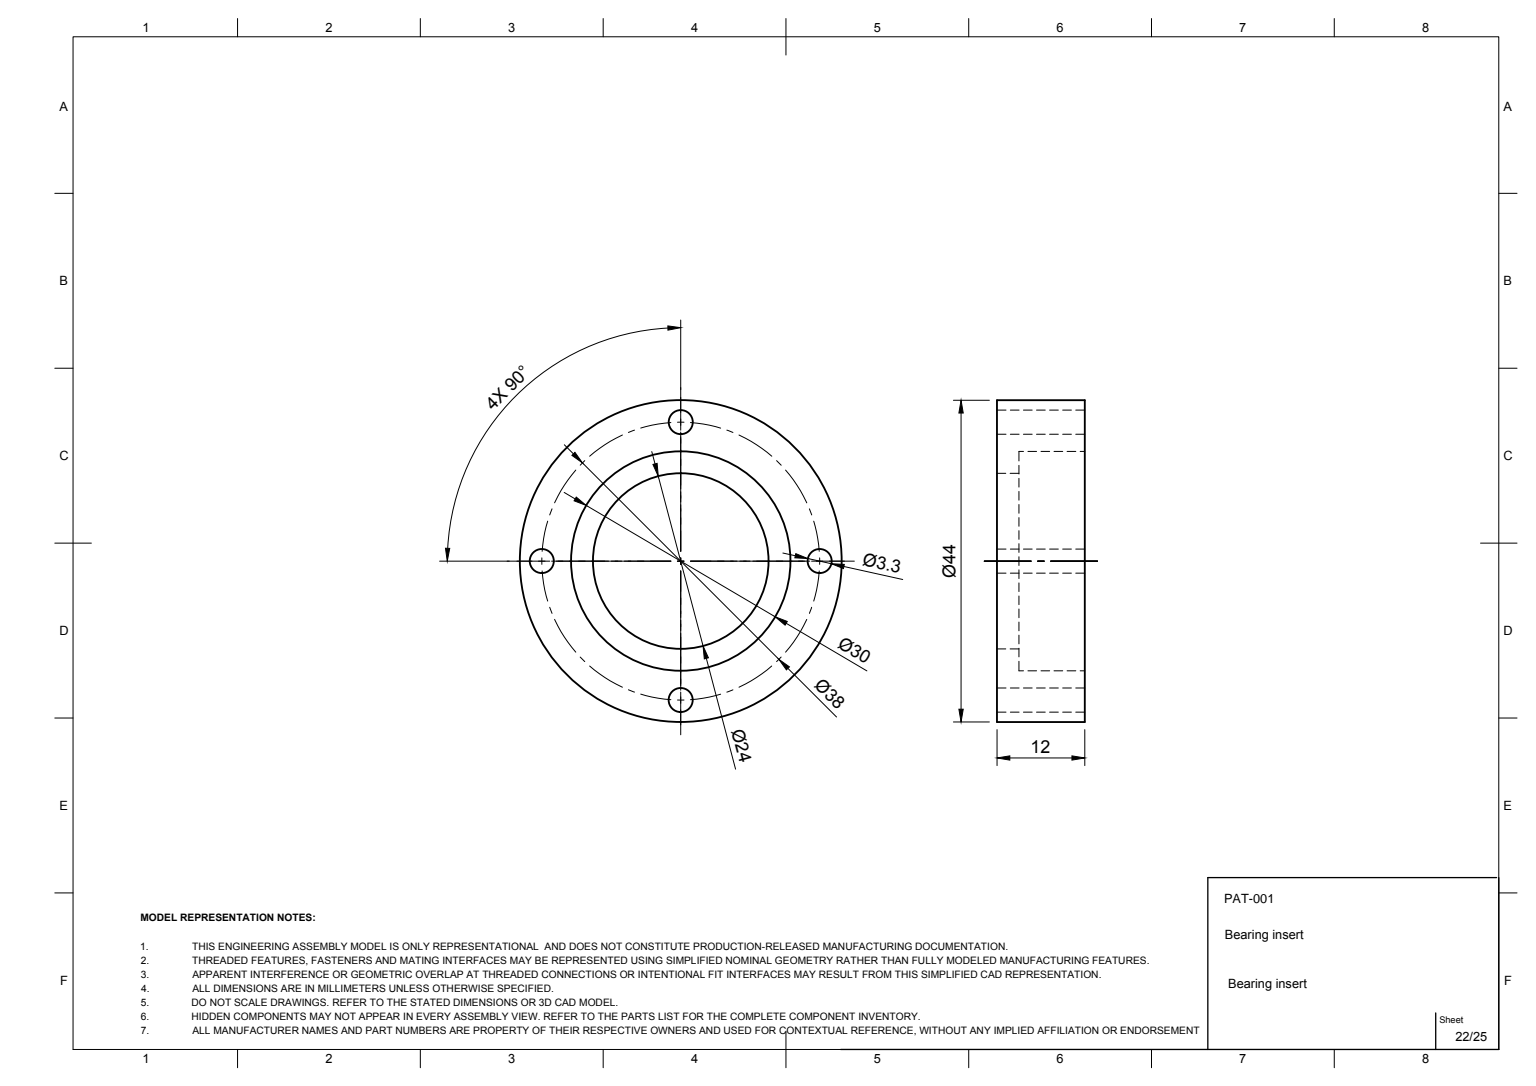
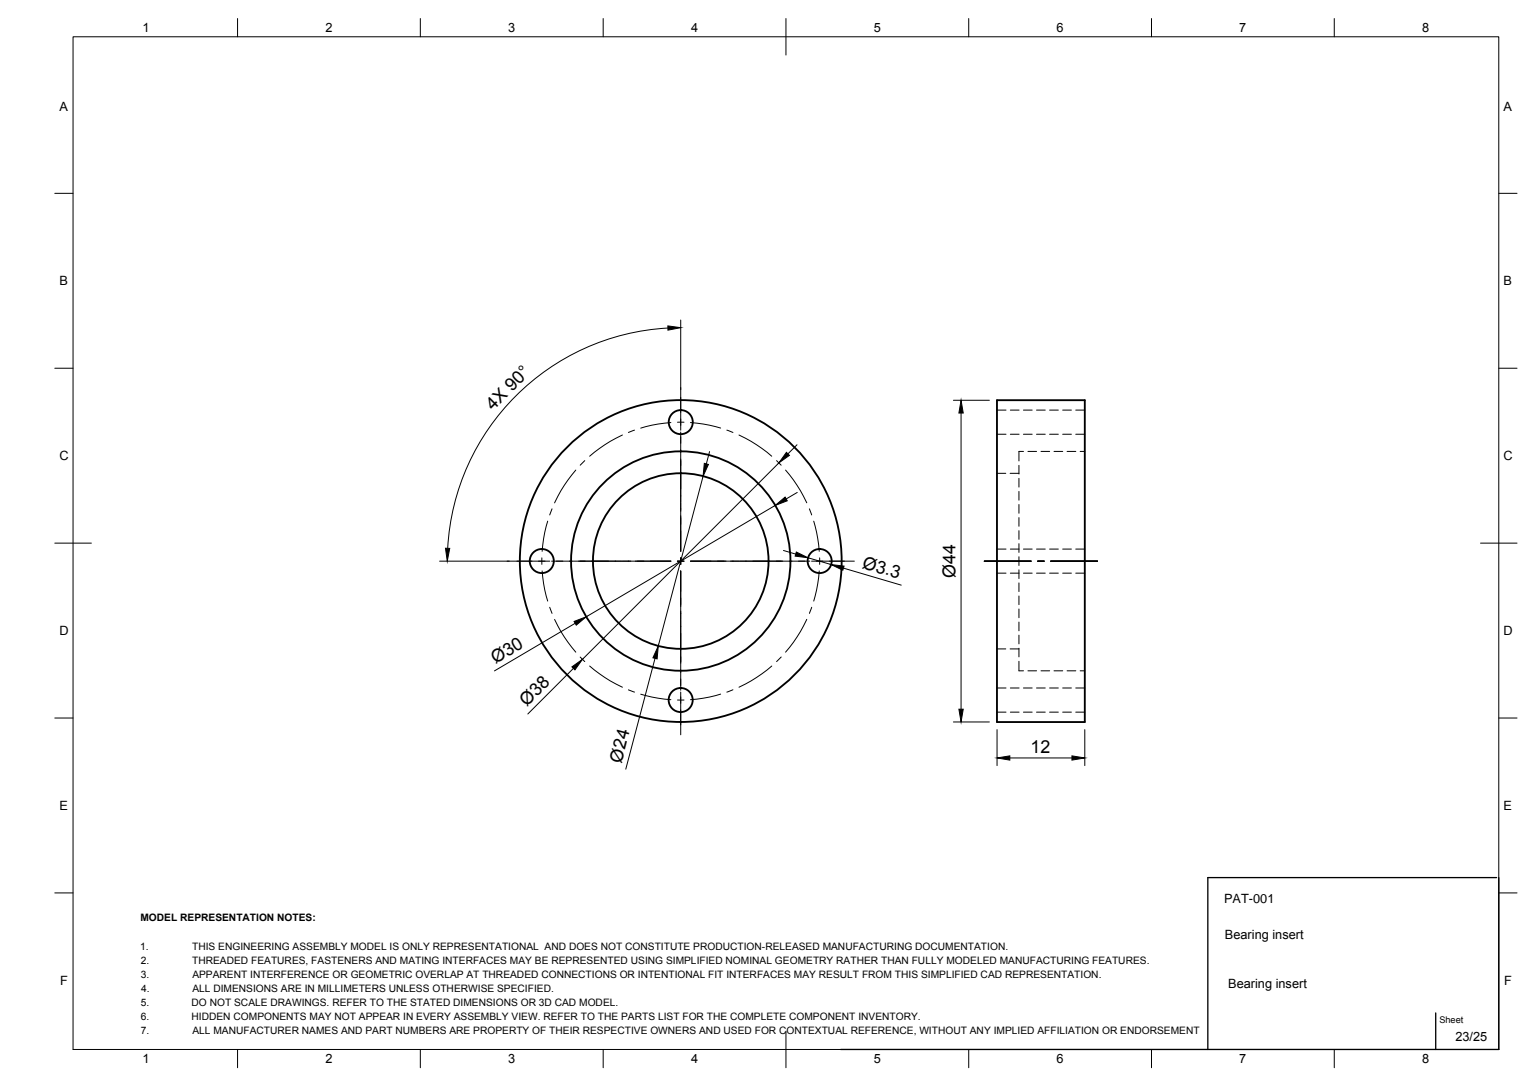
ISO-10303-21;
HEADER;
/* Generated by software containing ST-Developer
 * from STEP Tools, Inc. (www.steptools.com) 
 */

FILE_DESCRIPTION(
/* description */ ('PAT-001'),
/* implementation_level */ '2;1');

FILE_NAME(
/* name */ 'Bearing insert.step',
/* time_stamp */ '2026-10-29T17:07:15-07:00',
/* author */ (''),
/* organization */ (''),
/* preprocessor_version */ 'ST-DEVELOPER v20.2',
/* originating_system */ 'Autodesk Translation Framework v15.17.0.0',
/* authorisation */ '');

FILE_SCHEMA (('AUTOMOTIVE_DESIGN { 1 0 10303 214 3 1 1 }'));
ENDSEC;

DATA;
#10=MECHANICAL_DESIGN_GEOMETRIC_PRESENTATION_REPRESENTATION('',(#401),#9622);
#343=SHAPE_REPRESENTATION_RELATIONSHIP('SRR','None',#9768,#368);
#368=ADVANCED_BREP_SHAPE_REPRESENTATION('',(#433),#9617);
#401=STYLED_ITEM('',(#9962),#433);
#433=MANIFOLD_SOLID_BREP('Body1',#5227);
#493=FACE_BOUND('',#1320,.T.);
#494=FACE_BOUND('',#1324,.T.);
#495=FACE_BOUND('',#1325,.T.);
#496=FACE_BOUND('',#1326,.T.);
#497=FACE_BOUND('',#1327,.T.);
#498=FACE_BOUND('',#1328,.T.);
#499=FACE_BOUND('',#1330,.T.);
#500=FACE_BOUND('',#1331,.T.);
#501=FACE_BOUND('',#1332,.T.);
#502=FACE_BOUND('',#1333,.T.);
#503=FACE_BOUND('',#1334,.T.);
#694=PLANE('',#5963);
#695=PLANE('',#5970);
#696=PLANE('',#5971);
#962=FACE_OUTER_BOUND('',#1314,.T.);
#963=FACE_OUTER_BOUND('',#1315,.T.);
#964=FACE_OUTER_BOUND('',#1316,.T.);
#965=FACE_OUTER_BOUND('',#1317,.T.);
#966=FACE_OUTER_BOUND('',#1318,.T.);
#967=FACE_OUTER_BOUND('',#1319,.T.);
#968=FACE_OUTER_BOUND('',#1321,.T.);
#969=FACE_OUTER_BOUND('',#1322,.T.);
#970=FACE_OUTER_BOUND('',#1323,.T.);
#971=FACE_OUTER_BOUND('',#1329,.T.);
#1314=EDGE_LOOP('',(#4631,#4632,#4633,#4634));
#1315=EDGE_LOOP('',(#4635,#4636,#4637,#4638));
#1316=EDGE_LOOP('',(#4639,#4640,#4641,#4642));
#1317=EDGE_LOOP('',(#4643,#4644,#4645,#4646));
#1318=EDGE_LOOP('',(#4647,#4648,#4649,#4650));
#1319=EDGE_LOOP('',(#4651));
#1320=EDGE_LOOP('',(#4652));
#1321=EDGE_LOOP('',(#4653,#4654,#4655,#4656));
#1322=EDGE_LOOP('',(#4657,#4658,#4659,#4660));
#1323=EDGE_LOOP('',(#4661));
#1324=EDGE_LOOP('',(#4662));
#1325=EDGE_LOOP('',(#4663));
#1326=EDGE_LOOP('',(#4664));
#1327=EDGE_LOOP('',(#4665));
#1328=EDGE_LOOP('',(#4666));
#1329=EDGE_LOOP('',(#4667));
#1330=EDGE_LOOP('',(#4668));
#1331=EDGE_LOOP('',(#4669));
#1332=EDGE_LOOP('',(#4670));
#1333=EDGE_LOOP('',(#4671));
#1334=EDGE_LOOP('',(#4672));
#1757=LINE('',#9298,#2162);
#1758=LINE('',#9304,#2163);
#1759=LINE('',#9310,#2164);
#1760=LINE('',#9316,#2165);
#1761=LINE('',#9322,#2166);
#1762=LINE('',#9329,#2167);
#1763=LINE('',#9335,#2168);
#2162=VECTOR('',#7348,0.165);
#2163=VECTOR('',#7355,0.165);
#2164=VECTOR('',#7362,0.165);
#2165=VECTOR('',#7369,0.165);
#2166=VECTOR('',#7376,1.2);
#2167=VECTOR('',#7385,1.5);
#2168=VECTOR('',#7392,2.2);
#2368=CIRCLE('',#5949,0.165);
#2369=CIRCLE('',#5950,0.165);
#2370=CIRCLE('',#5952,0.165);
#2371=CIRCLE('',#5953,0.165);
#2372=CIRCLE('',#5955,0.165);
#2373=CIRCLE('',#5956,0.165);
#2374=CIRCLE('',#5958,0.165);
#2375=CIRCLE('',#5959,0.165);
#2376=CIRCLE('',#5961,1.2);
#2377=CIRCLE('',#5962,1.2);
#2378=CIRCLE('',#5964,1.5);
#2379=CIRCLE('',#5966,1.5);
#2380=CIRCLE('',#5968,2.2);
#2381=CIRCLE('',#5969,2.2);
#2798=VERTEX_POINT('',#9295);
#2799=VERTEX_POINT('',#9297);
#2800=VERTEX_POINT('',#9301);
#2801=VERTEX_POINT('',#9303);
#2802=VERTEX_POINT('',#9307);
#2803=VERTEX_POINT('',#9309);
#2804=VERTEX_POINT('',#9313);
#2805=VERTEX_POINT('',#9315);
#2806=VERTEX_POINT('',#9319);
#2807=VERTEX_POINT('',#9321);
#2808=VERTEX_POINT('',#9325);
#2809=VERTEX_POINT('',#9328);
#2810=VERTEX_POINT('',#9332);
#2811=VERTEX_POINT('',#9334);
#3419=EDGE_CURVE('',#2798,#2798,#2368,.T.);
#3420=EDGE_CURVE('',#2798,#2799,#1757,.T.);
#3421=EDGE_CURVE('',#2799,#2799,#2369,.T.);
#3422=EDGE_CURVE('',#2800,#2800,#2370,.T.);
#3423=EDGE_CURVE('',#2800,#2801,#1758,.T.);
#3424=EDGE_CURVE('',#2801,#2801,#2371,.T.);
#3425=EDGE_CURVE('',#2802,#2802,#2372,.T.);
#3426=EDGE_CURVE('',#2802,#2803,#1759,.T.);
#3427=EDGE_CURVE('',#2803,#2803,#2373,.T.);
#3428=EDGE_CURVE('',#2804,#2804,#2374,.T.);
#3429=EDGE_CURVE('',#2804,#2805,#1760,.T.);
#3430=EDGE_CURVE('',#2805,#2805,#2375,.T.);
#3431=EDGE_CURVE('',#2806,#2806,#2376,.T.);
#3432=EDGE_CURVE('',#2806,#2807,#1761,.T.);
#3433=EDGE_CURVE('',#2807,#2807,#2377,.T.);
#3434=EDGE_CURVE('',#2808,#2808,#2378,.T.);
#3435=EDGE_CURVE('',#2808,#2809,#1762,.T.);
#3436=EDGE_CURVE('',#2809,#2809,#2379,.T.);
#3437=EDGE_CURVE('',#2810,#2810,#2380,.T.);
#3438=EDGE_CURVE('',#2810,#2811,#1763,.T.);
#3439=EDGE_CURVE('',#2811,#2811,#2381,.T.);
#4631=ORIENTED_EDGE('',*,*,#3419,.F.);
#4632=ORIENTED_EDGE('',*,*,#3420,.T.);
#4633=ORIENTED_EDGE('',*,*,#3421,.F.);
#4634=ORIENTED_EDGE('',*,*,#3420,.F.);
#4635=ORIENTED_EDGE('',*,*,#3422,.F.);
#4636=ORIENTED_EDGE('',*,*,#3423,.T.);
#4637=ORIENTED_EDGE('',*,*,#3424,.F.);
#4638=ORIENTED_EDGE('',*,*,#3423,.F.);
#4639=ORIENTED_EDGE('',*,*,#3425,.F.);
#4640=ORIENTED_EDGE('',*,*,#3426,.T.);
#4641=ORIENTED_EDGE('',*,*,#3427,.F.);
#4642=ORIENTED_EDGE('',*,*,#3426,.F.);
#4643=ORIENTED_EDGE('',*,*,#3428,.F.);
#4644=ORIENTED_EDGE('',*,*,#3429,.T.);
#4645=ORIENTED_EDGE('',*,*,#3430,.F.);
#4646=ORIENTED_EDGE('',*,*,#3429,.F.);
#4647=ORIENTED_EDGE('',*,*,#3431,.F.);
#4648=ORIENTED_EDGE('',*,*,#3432,.T.);
#4649=ORIENTED_EDGE('',*,*,#3433,.T.);
#4650=ORIENTED_EDGE('',*,*,#3432,.F.);
#4651=ORIENTED_EDGE('',*,*,#3434,.F.);
#4652=ORIENTED_EDGE('',*,*,#3433,.F.);
#4653=ORIENTED_EDGE('',*,*,#3434,.T.);
#4654=ORIENTED_EDGE('',*,*,#3435,.T.);
#4655=ORIENTED_EDGE('',*,*,#3436,.T.);
#4656=ORIENTED_EDGE('',*,*,#3435,.F.);
#4657=ORIENTED_EDGE('',*,*,#3437,.F.);
#4658=ORIENTED_EDGE('',*,*,#3438,.T.);
#4659=ORIENTED_EDGE('',*,*,#3439,.T.);
#4660=ORIENTED_EDGE('',*,*,#3438,.F.);
#4661=ORIENTED_EDGE('',*,*,#3437,.T.);
#4662=ORIENTED_EDGE('',*,*,#3431,.T.);
#4663=ORIENTED_EDGE('',*,*,#3430,.T.);
#4664=ORIENTED_EDGE('',*,*,#3427,.T.);
#4665=ORIENTED_EDGE('',*,*,#3424,.T.);
#4666=ORIENTED_EDGE('',*,*,#3421,.T.);
#4667=ORIENTED_EDGE('',*,*,#3439,.F.);
#4668=ORIENTED_EDGE('',*,*,#3436,.F.);
#4669=ORIENTED_EDGE('',*,*,#3428,.T.);
#4670=ORIENTED_EDGE('',*,*,#3425,.T.);
#4671=ORIENTED_EDGE('',*,*,#3422,.T.);
#4672=ORIENTED_EDGE('',*,*,#3419,.T.);
#4878=CYLINDRICAL_SURFACE('',#5948,0.165);
#4879=CYLINDRICAL_SURFACE('',#5951,0.165);
#4880=CYLINDRICAL_SURFACE('',#5954,0.165);
#4881=CYLINDRICAL_SURFACE('',#5957,0.165);
#4882=CYLINDRICAL_SURFACE('',#5960,1.2);
#4883=CYLINDRICAL_SURFACE('',#5965,1.5);
#4884=CYLINDRICAL_SURFACE('',#5967,2.2);
#5149=ADVANCED_FACE('',(#962),#4878,.F.);
#5150=ADVANCED_FACE('',(#963),#4879,.F.);
#5151=ADVANCED_FACE('',(#964),#4880,.F.);
#5152=ADVANCED_FACE('',(#965),#4881,.F.);
#5153=ADVANCED_FACE('',(#966),#4882,.F.);
#5154=ADVANCED_FACE('',(#967,#493),#694,.F.);
#5155=ADVANCED_FACE('',(#968),#4883,.F.);
#5156=ADVANCED_FACE('',(#969),#4884,.T.);
#5157=ADVANCED_FACE('',(#970,#494,#495,#496,#497,#498),#695,.T.);
#5158=ADVANCED_FACE('',(#971,#499,#500,#501,#502,#503),#696,.F.);
#5227=CLOSED_SHELL('',(#5149,#5150,#5151,#5152,#5153,#5154,#5155,#5156,
#5157,#5158));
#5947=AXIS2_PLACEMENT_3D('',#9293,#7342,#7343);
#5948=AXIS2_PLACEMENT_3D('',#9294,#7344,#7345);
#5949=AXIS2_PLACEMENT_3D('',#9296,#7346,#7347);
#5950=AXIS2_PLACEMENT_3D('',#9299,#7349,#7350);
#5951=AXIS2_PLACEMENT_3D('',#9300,#7351,#7352);
#5952=AXIS2_PLACEMENT_3D('',#9302,#7353,#7354);
#5953=AXIS2_PLACEMENT_3D('',#9305,#7356,#7357);
#5954=AXIS2_PLACEMENT_3D('',#9306,#7358,#7359);
#5955=AXIS2_PLACEMENT_3D('',#9308,#7360,#7361);
#5956=AXIS2_PLACEMENT_3D('',#9311,#7363,#7364);
#5957=AXIS2_PLACEMENT_3D('',#9312,#7365,#7366);
#5958=AXIS2_PLACEMENT_3D('',#9314,#7367,#7368);
#5959=AXIS2_PLACEMENT_3D('',#9317,#7370,#7371);
#5960=AXIS2_PLACEMENT_3D('',#9318,#7372,#7373);
#5961=AXIS2_PLACEMENT_3D('',#9320,#7374,#7375);
#5962=AXIS2_PLACEMENT_3D('',#9323,#7377,#7378);
#5963=AXIS2_PLACEMENT_3D('',#9324,#7379,#7380);
#5964=AXIS2_PLACEMENT_3D('',#9326,#7381,#7382);
#5965=AXIS2_PLACEMENT_3D('',#9327,#7383,#7384);
#5966=AXIS2_PLACEMENT_3D('',#9330,#7386,#7387);
#5967=AXIS2_PLACEMENT_3D('',#9331,#7388,#7389);
#5968=AXIS2_PLACEMENT_3D('',#9333,#7390,#7391);
#5969=AXIS2_PLACEMENT_3D('',#9336,#7393,#7394);
#5970=AXIS2_PLACEMENT_3D('',#9337,#7395,#7396);
#5971=AXIS2_PLACEMENT_3D('',#9338,#7397,#7398);
#7342=DIRECTION('axis',(0.,0.,1.));
#7343=DIRECTION('refdir',(1.,0.,0.));
#7344=DIRECTION('center_axis',(0.,1.,0.));
#7345=DIRECTION('ref_axis',(1.,0.,0.));
#7346=DIRECTION('center_axis',(0.,1.,0.));
#7347=DIRECTION('ref_axis',(1.,0.,0.));
#7348=DIRECTION('',(0.,1.,0.));
#7349=DIRECTION('center_axis',(0.,-1.,0.));
#7350=DIRECTION('ref_axis',(1.,0.,0.));
#7351=DIRECTION('center_axis',(0.,1.,0.));
#7352=DIRECTION('ref_axis',(1.,0.,0.));
#7353=DIRECTION('center_axis',(0.,1.,0.));
#7354=DIRECTION('ref_axis',(1.,0.,0.));
#7355=DIRECTION('',(0.,1.,0.));
#7356=DIRECTION('center_axis',(0.,-1.,0.));
#7357=DIRECTION('ref_axis',(1.,0.,0.));
#7358=DIRECTION('center_axis',(0.,1.,0.));
#7359=DIRECTION('ref_axis',(1.,0.,0.));
#7360=DIRECTION('center_axis',(0.,1.,0.));
#7361=DIRECTION('ref_axis',(1.,0.,0.));
#7362=DIRECTION('',(0.,1.,0.));
#7363=DIRECTION('center_axis',(0.,-1.,0.));
#7364=DIRECTION('ref_axis',(1.,0.,0.));
#7365=DIRECTION('center_axis',(0.,1.,0.));
#7366=DIRECTION('ref_axis',(1.,0.,0.));
#7367=DIRECTION('center_axis',(0.,1.,0.));
#7368=DIRECTION('ref_axis',(1.,0.,0.));
#7369=DIRECTION('',(0.,1.,0.));
#7370=DIRECTION('center_axis',(0.,-1.,0.));
#7371=DIRECTION('ref_axis',(1.,0.,0.));
#7372=DIRECTION('center_axis',(0.,1.,0.));
#7373=DIRECTION('ref_axis',(1.,0.,0.));
#7374=DIRECTION('center_axis',(0.,-1.,0.));
#7375=DIRECTION('ref_axis',(1.,0.,0.));
#7376=DIRECTION('',(0.,-1.,0.));
#7377=DIRECTION('center_axis',(0.,-1.,0.));
#7378=DIRECTION('ref_axis',(1.,0.,0.));
#7379=DIRECTION('center_axis',(0.,1.,0.));
#7380=DIRECTION('ref_axis',(1.,0.,0.));
#7381=DIRECTION('center_axis',(0.,1.,0.));
#7382=DIRECTION('ref_axis',(1.,0.,0.));
#7383=DIRECTION('center_axis',(0.,1.,0.));
#7384=DIRECTION('ref_axis',(1.,0.,0.));
#7385=DIRECTION('',(0.,-1.,0.));
#7386=DIRECTION('center_axis',(0.,-1.,0.));
#7387=DIRECTION('ref_axis',(1.,0.,0.));
#7388=DIRECTION('center_axis',(0.,1.,0.));
#7389=DIRECTION('ref_axis',(1.,0.,0.));
#7390=DIRECTION('center_axis',(0.,1.,0.));
#7391=DIRECTION('ref_axis',(1.,0.,0.));
#7392=DIRECTION('',(0.,-1.,0.));
#7393=DIRECTION('center_axis',(0.,1.,0.));
#7394=DIRECTION('ref_axis',(1.,0.,0.));
#7395=DIRECTION('center_axis',(0.,1.,0.));
#7396=DIRECTION('ref_axis',(1.,0.,0.));
#7397=DIRECTION('center_axis',(0.,1.,0.));
#7398=DIRECTION('ref_axis',(1.,0.,0.));
#9293=CARTESIAN_POINT('',(0.,0.,0.));
#9294=CARTESIAN_POINT('Origin',(-1.9,-0.1,4.5));
#9295=CARTESIAN_POINT('',(-2.065,0.,4.5));
#9296=CARTESIAN_POINT('Origin',(-1.9,0.,4.5));
#9297=CARTESIAN_POINT('',(-2.065,1.2,4.5));
#9298=CARTESIAN_POINT('',(-2.065,-0.1,4.5));
#9299=CARTESIAN_POINT('Origin',(-1.9,1.2,4.5));
#9300=CARTESIAN_POINT('Origin',(1.16341445918999E-16,-0.1,6.4));
#9301=CARTESIAN_POINT('',(-0.165,0.,6.4));
#9302=CARTESIAN_POINT('Origin',(1.16341445918999E-16,0.,6.4));
#9303=CARTESIAN_POINT('',(-0.165,1.2,6.4));
#9304=CARTESIAN_POINT('',(-0.165,-0.1,6.4));
#9305=CARTESIAN_POINT('Origin',(1.16341445918999E-16,1.2,6.4));
#9306=CARTESIAN_POINT('Origin',(1.9,-0.1,4.5));
#9307=CARTESIAN_POINT('',(1.735,0.,4.5));
#9308=CARTESIAN_POINT('Origin',(1.9,0.,4.5));
#9309=CARTESIAN_POINT('',(1.735,1.2,4.5));
#9310=CARTESIAN_POINT('',(1.735,-0.1,4.5));
#9311=CARTESIAN_POINT('Origin',(1.9,1.2,4.5));
#9312=CARTESIAN_POINT('Origin',(-3.49024337756996E-16,-0.1,2.6));
#9313=CARTESIAN_POINT('',(-0.165,0.,2.6));
#9314=CARTESIAN_POINT('Origin',(-3.49024337756996E-16,0.,2.6));
#9315=CARTESIAN_POINT('',(-0.165,1.2,2.6));
#9316=CARTESIAN_POINT('',(-0.165,-0.1,2.6));
#9317=CARTESIAN_POINT('Origin',(-3.49024337756996E-16,1.2,2.6));
#9318=CARTESIAN_POINT('Origin',(0.,0.9,4.5));
#9319=CARTESIAN_POINT('',(-1.2,1.2,4.5));
#9320=CARTESIAN_POINT('Origin',(0.,1.2,4.5));
#9321=CARTESIAN_POINT('',(-1.2,0.9,4.5));
#9322=CARTESIAN_POINT('',(-1.2,0.9,4.5));
#9323=CARTESIAN_POINT('Origin',(0.,0.9,4.5));
#9324=CARTESIAN_POINT('Origin',(0.,0.9,4.5));
#9325=CARTESIAN_POINT('',(-1.5,0.9,4.5));
#9326=CARTESIAN_POINT('Origin',(0.,0.9,4.5));
#9327=CARTESIAN_POINT('Origin',(0.,0.,4.5));
#9328=CARTESIAN_POINT('',(-1.5,0.,4.5));
#9329=CARTESIAN_POINT('',(-1.5,0.,4.5));
#9330=CARTESIAN_POINT('Origin',(0.,0.,4.5));
#9331=CARTESIAN_POINT('Origin',(0.,0.,4.5));
#9332=CARTESIAN_POINT('',(-2.2,1.2,4.5));
#9333=CARTESIAN_POINT('Origin',(0.,1.2,4.5));
#9334=CARTESIAN_POINT('',(-2.2,0.,4.5));
#9335=CARTESIAN_POINT('',(-2.2,0.,4.5));
#9336=CARTESIAN_POINT('Origin',(0.,0.,4.5));
#9337=CARTESIAN_POINT('Origin',(0.,1.2,4.5));
#9338=CARTESIAN_POINT('Origin',(0.,0.,4.5));
#9587=UNCERTAINTY_MEASURE_WITH_UNIT(LENGTH_MEASURE(0.001),#9623,
'DISTANCE_ACCURACY_VALUE',
'Maximum model space distance between geometric entities at asserted c
onnectivities');
#9592=UNCERTAINTY_MEASURE_WITH_UNIT(LENGTH_MEASURE(0.001),#9623,
'DISTANCE_ACCURACY_VALUE',
'Maximum model space distance between geometric entities at asserted c
onnectivities');
#9617=(
GEOMETRIC_REPRESENTATION_CONTEXT(3)
GLOBAL_UNCERTAINTY_ASSIGNED_CONTEXT((#9587))
GLOBAL_UNIT_ASSIGNED_CONTEXT((#9623,#9625,#9626))
REPRESENTATION_CONTEXT('','3D')
);
#9622=(
GEOMETRIC_REPRESENTATION_CONTEXT(3)
GLOBAL_UNCERTAINTY_ASSIGNED_CONTEXT((#9592))
GLOBAL_UNIT_ASSIGNED_CONTEXT((#9623,#9625,#9626))
REPRESENTATION_CONTEXT('','3D')
);
#9623=(
LENGTH_UNIT()
NAMED_UNIT(*)
SI_UNIT(.CENTI.,.METRE.)
);
#9625=(
NAMED_UNIT(*)
PLANE_ANGLE_UNIT()
SI_UNIT($,.RADIAN.)
);
#9626=(
NAMED_UNIT(*)
SI_UNIT($,.STERADIAN.)
SOLID_ANGLE_UNIT()
);
#9651=SHAPE_DEFINITION_REPRESENTATION(#9685,#9768);
#9685=PRODUCT_DEFINITION_SHAPE('',$,#9798);
#9768=SHAPE_REPRESENTATION('',(#5947),#9617);
#9773=PRODUCT_DEFINITION_CONTEXT('part definition',#9862,'design');
#9798=PRODUCT_DEFINITION('Bearing insert','Bearing insert',#9827,#9773);
#9827=PRODUCT_DEFINITION_FORMATION('',$,#9888);
#9862=APPLICATION_CONTEXT(
'Core Data for Automotive Mechanical Design Process');
#9863=PRODUCT_CONTEXT('part definition',#9862,'mechanical');
#9888=PRODUCT('Bearing insert','Bearing insert','Bearing insert',(#9863));
#9956=COLOUR_RGB('Grey',0.48,0.52,0.57);
#9957=FILL_AREA_STYLE_COLOUR('',#9956);
#9958=FILL_AREA_STYLE('',(#9957));
#9959=SURFACE_STYLE_FILL_AREA(#9958);
#9960=SURFACE_SIDE_STYLE('',(#9959));
#9961=SURFACE_STYLE_USAGE(.BOTH.,#9960);
#9962=PRESENTATION_STYLE_ASSIGNMENT((#9961));
ENDSEC;
END-ISO-10303-21;
